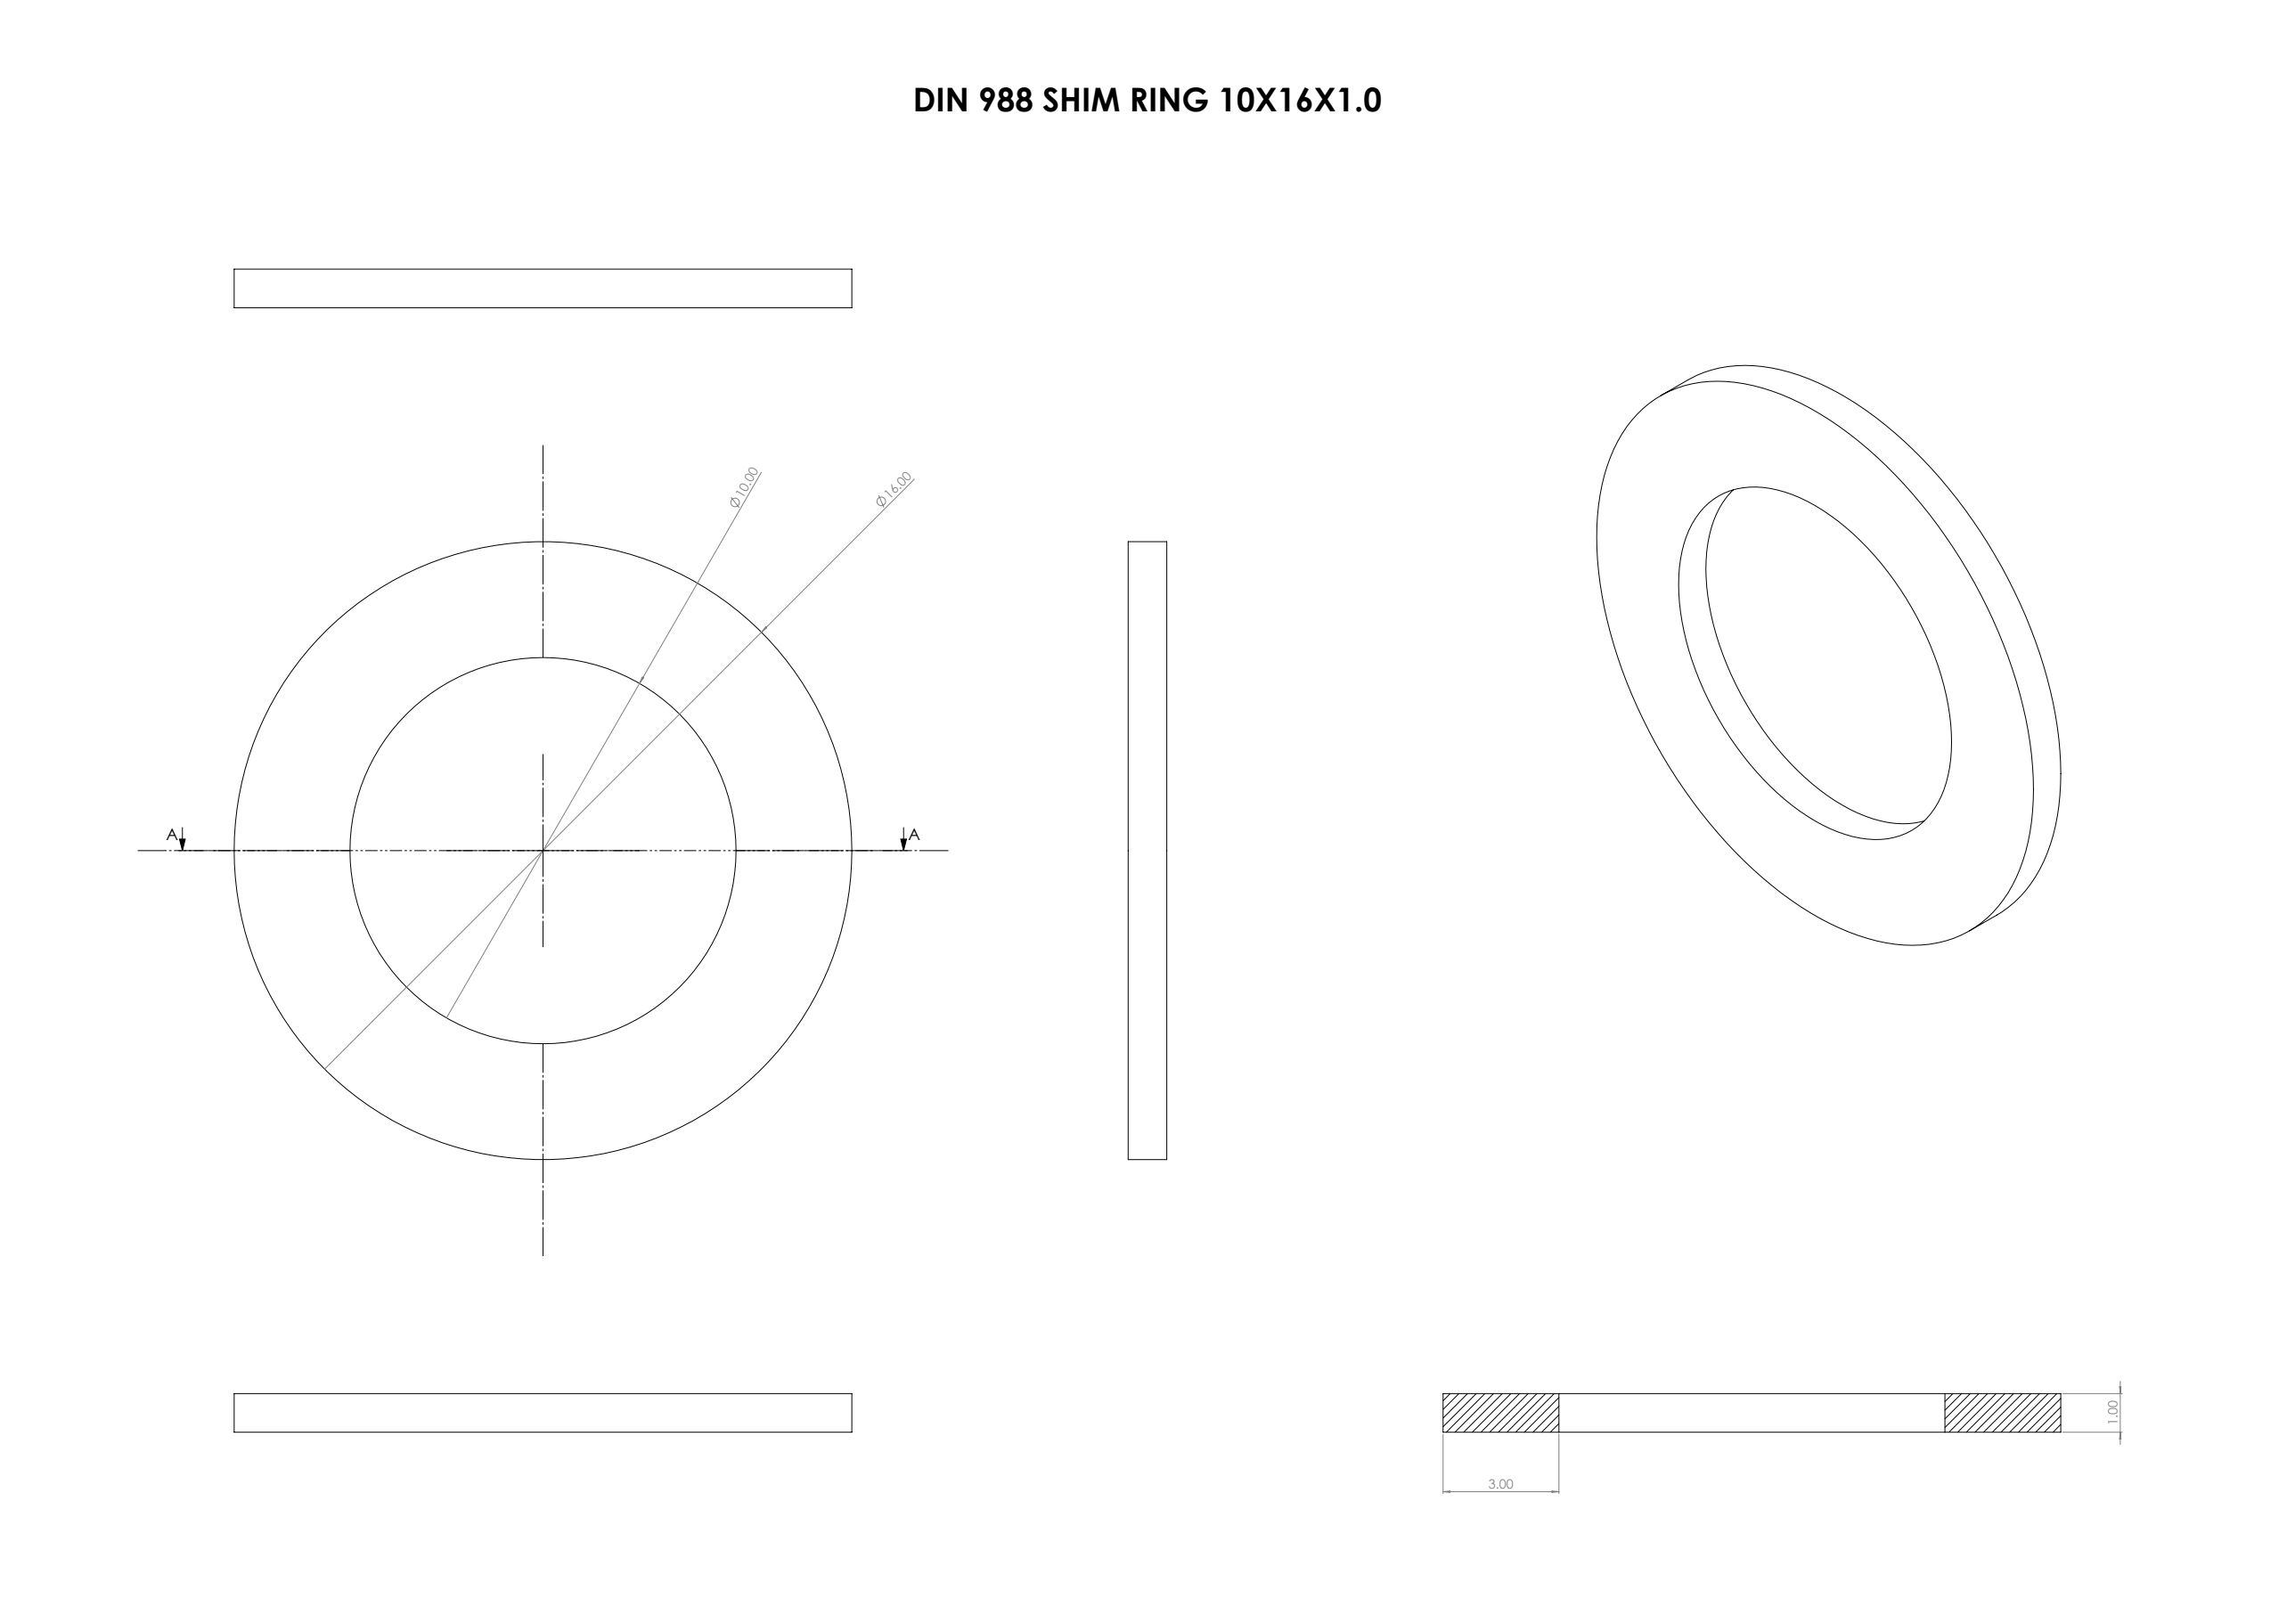
ISO-10303-21;
HEADER;
/* Generated by software containing ST-Developer
 * from STEP Tools, Inc. (www.steptools.com) 
 */

FILE_DESCRIPTION(
/* description */ (''),
/* implementation_level */ '2;1');

FILE_NAME(
/* name */ 
'06_DIN_988_Shim_Ring_10x16x1.0.step',
/* time_stamp */ '2026-10-22T00:21:42-07:00',
/* author */ (''),
/* organization */ (''),
/* preprocessor_version */ 'ST-DEVELOPER v20.2',
/* originating_system */ 'Autodesk Translation Framework v15.15.0.0',
/* authorisation */ '');

FILE_SCHEMA (('AUTOMOTIVE_DESIGN { 1 0 10303 214 3 1 1 }'));
ENDSEC;

DATA;
#10=MECHANICAL_DESIGN_GEOMETRIC_PRESENTATION_REPRESENTATION('',(#210),#31638);
#188=SHAPE_REPRESENTATION_RELATIONSHIP('SRR','None',#31710,#199);
#199=ADVANCED_BREP_SHAPE_REPRESENTATION('',(#221),#31632);
#210=STYLED_ITEM('',(#31823),#221);
#221=MANIFOLD_SOLID_BREP('Shim ring',#12485);
#287=CYLINDRICAL_SURFACE('',#13097,0.5);
#288=CYLINDRICAL_SURFACE('',#13102,0.8);
#1390=FACE_BOUND('',#2946,.T.);
#1391=FACE_BOUND('',#2949,.T.);
#1645=CIRCLE('',#13098,0.5);
#1646=CIRCLE('',#13099,0.5);
#1647=CIRCLE('',#13101,0.8);
#1648=CIRCLE('',#13103,0.8);
#2200=FACE_OUTER_BOUND('',#2944,.T.);
#2201=FACE_OUTER_BOUND('',#2945,.T.);
#2202=FACE_OUTER_BOUND('',#2947,.T.);
#2203=FACE_OUTER_BOUND('',#2948,.T.);
#2944=EDGE_LOOP('',(#9909,#9910,#9911,#9912));
#2945=EDGE_LOOP('',(#9913));
#2946=EDGE_LOOP('',(#9914));
#2947=EDGE_LOOP('',(#9915,#9916,#9917,#9918));
#2948=EDGE_LOOP('',(#9919));
#2949=EDGE_LOOP('',(#9920));
#3552=LINE('',#25734,#4257);
#3553=LINE('',#25742,#4258);
#4257=VECTOR('',#14872,0.5);
#4258=VECTOR('',#14883,0.8);
#5397=VERTEX_POINT('',#25731);
#5398=VERTEX_POINT('',#25733);
#5399=VERTEX_POINT('',#25737);
#5400=VERTEX_POINT('',#25740);
#6966=EDGE_CURVE('',#5397,#5397,#1645,.T.);
#6967=EDGE_CURVE('',#5397,#5398,#3552,.T.);
#6968=EDGE_CURVE('',#5398,#5398,#1646,.T.);
#6969=EDGE_CURVE('',#5399,#5399,#1647,.T.);
#6970=EDGE_CURVE('',#5400,#5400,#1648,.T.);
#6971=EDGE_CURVE('',#5400,#5399,#3553,.T.);
#9909=ORIENTED_EDGE('',*,*,#6966,.T.);
#9910=ORIENTED_EDGE('',*,*,#6967,.T.);
#9911=ORIENTED_EDGE('',*,*,#6968,.F.);
#9912=ORIENTED_EDGE('',*,*,#6967,.F.);
#9913=ORIENTED_EDGE('',*,*,#6969,.F.);
#9914=ORIENTED_EDGE('',*,*,#6968,.T.);
#9915=ORIENTED_EDGE('',*,*,#6970,.F.);
#9916=ORIENTED_EDGE('',*,*,#6971,.T.);
#9917=ORIENTED_EDGE('',*,*,#6969,.T.);
#9918=ORIENTED_EDGE('',*,*,#6971,.F.);
#9919=ORIENTED_EDGE('',*,*,#6970,.T.);
#9920=ORIENTED_EDGE('',*,*,#6966,.F.);
#11581=PLANE('',#13100);
#11582=PLANE('',#13104);
#12167=ADVANCED_FACE('',(#2200),#287,.F.);
#12168=ADVANCED_FACE('',(#2201,#1390),#11581,.T.);
#12169=ADVANCED_FACE('',(#2202),#288,.T.);
#12170=ADVANCED_FACE('',(#2203,#1391),#11582,.T.);
#12485=CLOSED_SHELL('',(#12167,#12168,#12169,#12170));
#13096=AXIS2_PLACEMENT_3D('',#25729,#14866,#14867);
#13097=AXIS2_PLACEMENT_3D('',#25730,#14868,#14869);
#13098=AXIS2_PLACEMENT_3D('',#25732,#14870,#14871);
#13099=AXIS2_PLACEMENT_3D('',#25735,#14873,#14874);
#13100=AXIS2_PLACEMENT_3D('',#25736,#14875,#14876);
#13101=AXIS2_PLACEMENT_3D('',#25738,#14877,#14878);
#13102=AXIS2_PLACEMENT_3D('',#25739,#14879,#14880);
#13103=AXIS2_PLACEMENT_3D('',#25741,#14881,#14882);
#13104=AXIS2_PLACEMENT_3D('',#25743,#14884,#14885);
#14866=DIRECTION('axis',(0.,0.,1.));
#14867=DIRECTION('refdir',(1.,0.,0.));
#14868=DIRECTION('center_axis',(0.,0.,1.));
#14869=DIRECTION('ref_axis',(1.,0.,0.));
#14870=DIRECTION('center_axis',(0.,0.,1.));
#14871=DIRECTION('ref_axis',(1.,0.,0.));
#14872=DIRECTION('',(0.,0.,-1.));
#14873=DIRECTION('center_axis',(0.,0.,1.));
#14874=DIRECTION('ref_axis',(1.,0.,0.));
#14875=DIRECTION('center_axis',(0.,0.,-1.));
#14876=DIRECTION('ref_axis',(-1.,0.,0.));
#14877=DIRECTION('center_axis',(0.,0.,1.));
#14878=DIRECTION('ref_axis',(1.,0.,0.));
#14879=DIRECTION('center_axis',(0.,0.,1.));
#14880=DIRECTION('ref_axis',(1.,0.,0.));
#14881=DIRECTION('center_axis',(0.,0.,1.));
#14882=DIRECTION('ref_axis',(1.,0.,0.));
#14883=DIRECTION('',(0.,0.,-1.));
#14884=DIRECTION('center_axis',(0.,0.,1.));
#14885=DIRECTION('ref_axis',(1.,0.,0.));
#25729=CARTESIAN_POINT('',(0.,0.,0.));
#25730=CARTESIAN_POINT('Origin',(0.,0.,2.65));
#25731=CARTESIAN_POINT('',(-0.5,-6.12323399573677E-17,2.7));
#25732=CARTESIAN_POINT('Origin',(0.,0.,2.7));
#25733=CARTESIAN_POINT('',(-0.5,-6.12323399573677E-17,2.6));
#25734=CARTESIAN_POINT('',(-0.5,-6.12323399573677E-17,2.65));
#25735=CARTESIAN_POINT('Origin',(0.,0.,2.6));
#25736=CARTESIAN_POINT('Origin',(0.8,0.,2.6));
#25737=CARTESIAN_POINT('',(-0.8,-9.79717439317883E-17,2.6));
#25738=CARTESIAN_POINT('Origin',(0.,0.,2.6));
#25739=CARTESIAN_POINT('Origin',(0.,0.,2.65));
#25740=CARTESIAN_POINT('',(-0.8,-9.79717439317883E-17,2.7));
#25741=CARTESIAN_POINT('Origin',(0.,0.,2.7));
#25742=CARTESIAN_POINT('',(-0.8,-9.79717439317883E-17,2.65));
#25743=CARTESIAN_POINT('Origin',(0.5,0.,2.7));
#31619=UNCERTAINTY_MEASURE_WITH_UNIT(LENGTH_MEASURE(0.001),#31639,
'DISTANCE_ACCURACY_VALUE',
'Maximum model space distance between geometric entities at asserted c
onnectivities');
#31625=UNCERTAINTY_MEASURE_WITH_UNIT(LENGTH_MEASURE(0.001),#31639,
'DISTANCE_ACCURACY_VALUE',
'Maximum model space distance between geometric entities at asserted c
onnectivities');
#31632=(
GEOMETRIC_REPRESENTATION_CONTEXT(3)
GLOBAL_UNCERTAINTY_ASSIGNED_CONTEXT((#31619))
GLOBAL_UNIT_ASSIGNED_CONTEXT((#31639,#31641,#31642))
REPRESENTATION_CONTEXT('','3D')
);
#31638=(
GEOMETRIC_REPRESENTATION_CONTEXT(3)
GLOBAL_UNCERTAINTY_ASSIGNED_CONTEXT((#31625))
GLOBAL_UNIT_ASSIGNED_CONTEXT((#31639,#31641,#31642))
REPRESENTATION_CONTEXT('','3D')
);
#31639=(
LENGTH_UNIT()
NAMED_UNIT(*)
SI_UNIT(.CENTI.,.METRE.)
);
#31641=(
NAMED_UNIT(*)
PLANE_ANGLE_UNIT()
SI_UNIT($,.RADIAN.)
);
#31642=(
NAMED_UNIT(*)
SI_UNIT($,.STERADIAN.)
SOLID_ANGLE_UNIT()
);
#31649=SHAPE_DEFINITION_REPRESENTATION(#31661,#31710);
#31661=PRODUCT_DEFINITION_SHAPE('',$,#31723);
#31710=SHAPE_REPRESENTATION('',(#13096),#31632);
#31716=PRODUCT_DEFINITION_CONTEXT('part definition',#31754,'design');
#31723=PRODUCT_DEFINITION('2026-10-22-02-42-21-610',
'06_DIN_988_Shim_Ring_10x16x1.0',#31735,#31716);
#31735=PRODUCT_DEFINITION_FORMATION('',$,#31762);
#31754=APPLICATION_CONTEXT(
'Core Data for Automotive Mechanical Design Process');
#31755=PRODUCT_CONTEXT('part definition',#31754,'mechanical');
#31762=PRODUCT('2026-10-22-02-42-21-610',
'06_DIN_988_Shim_Ring_10x16x1.0',$,(#31755));
#31817=COLOUR_RGB('Sky Blue',0.24,0.69,0.87);
#31818=FILL_AREA_STYLE_COLOUR('',#31817);
#31819=FILL_AREA_STYLE('',(#31818));
#31820=SURFACE_STYLE_FILL_AREA(#31819);
#31821=SURFACE_SIDE_STYLE('',(#31820));
#31822=SURFACE_STYLE_USAGE(.BOTH.,#31821);
#31823=PRESENTATION_STYLE_ASSIGNMENT((#31822));
ENDSEC;
END-ISO-10303-21;
